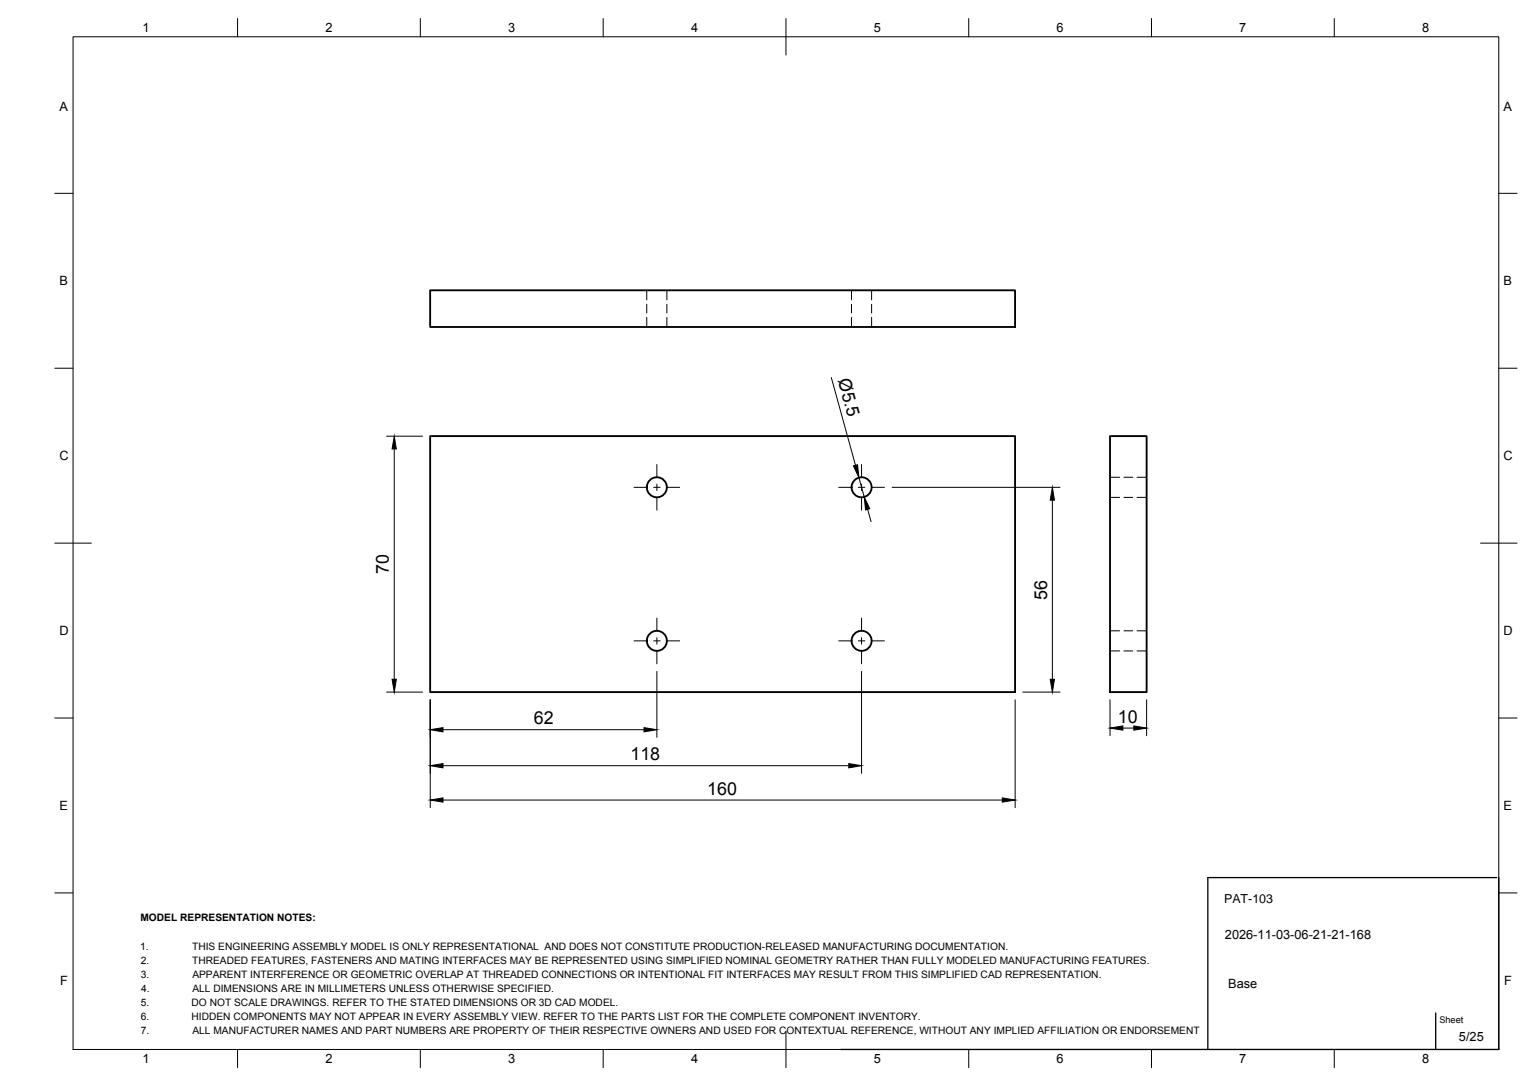
ISO-10303-21;
HEADER;
/* Generated by software containing ST-Developer
 * from STEP Tools, Inc. (www.steptools.com) 
 */

FILE_DESCRIPTION(
/* description */ ('Telescoping shaft support with lock collar'),
/* implementation_level */ '2;1');

FILE_NAME(
/* name */ 'Base.step',
/* time_stamp */ '2026-10-27T10:48:51-07:00',
/* author */ (''),
/* organization */ (''),
/* preprocessor_version */ 'ST-DEVELOPER v20.2',
/* originating_system */ 'Autodesk Translation Framework v15.17.0.0',
/* authorisation */ '');

FILE_SCHEMA (('AUTOMOTIVE_DESIGN { 1 0 10303 214 3 1 1 }'));
ENDSEC;

DATA;
#10=MECHANICAL_DESIGN_GEOMETRIC_PRESENTATION_REPRESENTATION('',(#241),#7349);
#201=SHAPE_REPRESENTATION_RELATIONSHIP('SRR','None',#7443,#221);
#221=ADVANCED_BREP_SHAPE_REPRESENTATION('',(#261),#7327);
#241=STYLED_ITEM('',(#7606),#261);
#261=MANIFOLD_SOLID_BREP('Body1',#3964);
#279=FACE_BOUND('',#730,.T.);
#280=FACE_BOUND('',#731,.T.);
#281=FACE_BOUND('',#732,.T.);
#282=FACE_BOUND('',#733,.T.);
#283=FACE_BOUND('',#735,.T.);
#284=FACE_BOUND('',#736,.T.);
#285=FACE_BOUND('',#737,.T.);
#286=FACE_BOUND('',#738,.T.);
#359=PLANE('',#4222);
#360=PLANE('',#4223);
#361=PLANE('',#4224);
#362=PLANE('',#4225);
#363=PLANE('',#4226);
#364=PLANE('',#4227);
#495=FACE_OUTER_BOUND('',#721,.T.);
#496=FACE_OUTER_BOUND('',#722,.T.);
#497=FACE_OUTER_BOUND('',#723,.T.);
#498=FACE_OUTER_BOUND('',#724,.T.);
#499=FACE_OUTER_BOUND('',#725,.T.);
#500=FACE_OUTER_BOUND('',#726,.T.);
#501=FACE_OUTER_BOUND('',#727,.T.);
#502=FACE_OUTER_BOUND('',#728,.T.);
#503=FACE_OUTER_BOUND('',#729,.T.);
#504=FACE_OUTER_BOUND('',#734,.T.);
#721=EDGE_LOOP('',(#2642,#2643,#2644,#2645));
#722=EDGE_LOOP('',(#2646,#2647,#2648,#2649));
#723=EDGE_LOOP('',(#2650,#2651,#2652,#2653));
#724=EDGE_LOOP('',(#2654,#2655,#2656,#2657));
#725=EDGE_LOOP('',(#2658,#2659,#2660,#2661));
#726=EDGE_LOOP('',(#2662,#2663,#2664,#2665));
#727=EDGE_LOOP('',(#2666,#2667,#2668,#2669));
#728=EDGE_LOOP('',(#2670,#2671,#2672,#2673));
#729=EDGE_LOOP('',(#2674,#2675,#2676,#2677));
#730=EDGE_LOOP('',(#2678));
#731=EDGE_LOOP('',(#2679));
#732=EDGE_LOOP('',(#2680));
#733=EDGE_LOOP('',(#2681));
#734=EDGE_LOOP('',(#2682,#2683,#2684,#2685));
#735=EDGE_LOOP('',(#2686));
#736=EDGE_LOOP('',(#2687));
#737=EDGE_LOOP('',(#2688));
#738=EDGE_LOOP('',(#2689));
#1027=LINE('',#5994,#1307);
#1028=LINE('',#6000,#1308);
#1029=LINE('',#6006,#1309);
#1030=LINE('',#6012,#1310);
#1031=LINE('',#6017,#1311);
#1032=LINE('',#6019,#1312);
#1033=LINE('',#6021,#1313);
#1034=LINE('',#6022,#1314);
#1035=LINE('',#6025,#1315);
#1036=LINE('',#6027,#1316);
#1037=LINE('',#6028,#1317);
#1038=LINE('',#6031,#1318);
#1039=LINE('',#6033,#1319);
#1040=LINE('',#6034,#1320);
#1041=LINE('',#6036,#1321);
#1042=LINE('',#6037,#1322);
#1307=VECTOR('',#4717,0.274999999999999);
#1308=VECTOR('',#4724,0.275);
#1309=VECTOR('',#4731,0.275);
#1310=VECTOR('',#4738,0.274999999999999);
#1311=VECTOR('',#4743,1.);
#1312=VECTOR('',#4744,1.);
#1313=VECTOR('',#4745,1.);
#1314=VECTOR('',#4746,1.);
#1315=VECTOR('',#4749,1.);
#1316=VECTOR('',#4750,1.);
#1317=VECTOR('',#4751,1.);
#1318=VECTOR('',#4754,1.);
#1319=VECTOR('',#4755,1.);
#1320=VECTOR('',#4756,1.);
#1321=VECTOR('',#4759,1.);
#1322=VECTOR('',#4760,1.);
#1587=CIRCLE('',#4211,0.274999999999999);
#1588=CIRCLE('',#4212,0.274999999999999);
#1589=CIRCLE('',#4214,0.275);
#1590=CIRCLE('',#4215,0.275);
#1591=CIRCLE('',#4217,0.275);
#1592=CIRCLE('',#4218,0.275);
#1593=CIRCLE('',#4220,0.274999999999999);
#1594=CIRCLE('',#4221,0.274999999999999);
#1798=VERTEX_POINT('',#5991);
#1799=VERTEX_POINT('',#5993);
#1800=VERTEX_POINT('',#5997);
#1801=VERTEX_POINT('',#5999);
#1802=VERTEX_POINT('',#6003);
#1803=VERTEX_POINT('',#6005);
#1804=VERTEX_POINT('',#6009);
#1805=VERTEX_POINT('',#6011);
#1806=VERTEX_POINT('',#6015);
#1807=VERTEX_POINT('',#6016);
#1808=VERTEX_POINT('',#6018);
#1809=VERTEX_POINT('',#6020);
#1810=VERTEX_POINT('',#6024);
#1811=VERTEX_POINT('',#6026);
#1812=VERTEX_POINT('',#6030);
#1813=VERTEX_POINT('',#6032);
#2133=EDGE_CURVE('',#1798,#1798,#1587,.T.);
#2134=EDGE_CURVE('',#1798,#1799,#1027,.T.);
#2135=EDGE_CURVE('',#1799,#1799,#1588,.T.);
#2136=EDGE_CURVE('',#1800,#1800,#1589,.T.);
#2137=EDGE_CURVE('',#1800,#1801,#1028,.T.);
#2138=EDGE_CURVE('',#1801,#1801,#1590,.T.);
#2139=EDGE_CURVE('',#1802,#1802,#1591,.T.);
#2140=EDGE_CURVE('',#1802,#1803,#1029,.T.);
#2141=EDGE_CURVE('',#1803,#1803,#1592,.T.);
#2142=EDGE_CURVE('',#1804,#1804,#1593,.T.);
#2143=EDGE_CURVE('',#1804,#1805,#1030,.T.);
#2144=EDGE_CURVE('',#1805,#1805,#1594,.T.);
#2145=EDGE_CURVE('',#1806,#1807,#1031,.T.);
#2146=EDGE_CURVE('',#1807,#1808,#1032,.T.);
#2147=EDGE_CURVE('',#1809,#1808,#1033,.T.);
#2148=EDGE_CURVE('',#1806,#1809,#1034,.T.);
#2149=EDGE_CURVE('',#1810,#1806,#1035,.T.);
#2150=EDGE_CURVE('',#1811,#1809,#1036,.T.);
#2151=EDGE_CURVE('',#1810,#1811,#1037,.T.);
#2152=EDGE_CURVE('',#1812,#1810,#1038,.T.);
#2153=EDGE_CURVE('',#1813,#1811,#1039,.T.);
#2154=EDGE_CURVE('',#1812,#1813,#1040,.T.);
#2155=EDGE_CURVE('',#1807,#1812,#1041,.T.);
#2156=EDGE_CURVE('',#1808,#1813,#1042,.T.);
#2642=ORIENTED_EDGE('',*,*,#2133,.F.);
#2643=ORIENTED_EDGE('',*,*,#2134,.T.);
#2644=ORIENTED_EDGE('',*,*,#2135,.F.);
#2645=ORIENTED_EDGE('',*,*,#2134,.F.);
#2646=ORIENTED_EDGE('',*,*,#2136,.F.);
#2647=ORIENTED_EDGE('',*,*,#2137,.T.);
#2648=ORIENTED_EDGE('',*,*,#2138,.F.);
#2649=ORIENTED_EDGE('',*,*,#2137,.F.);
#2650=ORIENTED_EDGE('',*,*,#2139,.F.);
#2651=ORIENTED_EDGE('',*,*,#2140,.T.);
#2652=ORIENTED_EDGE('',*,*,#2141,.F.);
#2653=ORIENTED_EDGE('',*,*,#2140,.F.);
#2654=ORIENTED_EDGE('',*,*,#2142,.F.);
#2655=ORIENTED_EDGE('',*,*,#2143,.T.);
#2656=ORIENTED_EDGE('',*,*,#2144,.F.);
#2657=ORIENTED_EDGE('',*,*,#2143,.F.);
#2658=ORIENTED_EDGE('',*,*,#2145,.T.);
#2659=ORIENTED_EDGE('',*,*,#2146,.T.);
#2660=ORIENTED_EDGE('',*,*,#2147,.F.);
#2661=ORIENTED_EDGE('',*,*,#2148,.F.);
#2662=ORIENTED_EDGE('',*,*,#2149,.T.);
#2663=ORIENTED_EDGE('',*,*,#2148,.T.);
#2664=ORIENTED_EDGE('',*,*,#2150,.F.);
#2665=ORIENTED_EDGE('',*,*,#2151,.F.);
#2666=ORIENTED_EDGE('',*,*,#2152,.T.);
#2667=ORIENTED_EDGE('',*,*,#2151,.T.);
#2668=ORIENTED_EDGE('',*,*,#2153,.F.);
#2669=ORIENTED_EDGE('',*,*,#2154,.F.);
#2670=ORIENTED_EDGE('',*,*,#2155,.T.);
#2671=ORIENTED_EDGE('',*,*,#2154,.T.);
#2672=ORIENTED_EDGE('',*,*,#2156,.F.);
#2673=ORIENTED_EDGE('',*,*,#2146,.F.);
#2674=ORIENTED_EDGE('',*,*,#2156,.T.);
#2675=ORIENTED_EDGE('',*,*,#2153,.T.);
#2676=ORIENTED_EDGE('',*,*,#2150,.T.);
#2677=ORIENTED_EDGE('',*,*,#2147,.T.);
#2678=ORIENTED_EDGE('',*,*,#2135,.T.);
#2679=ORIENTED_EDGE('',*,*,#2138,.T.);
#2680=ORIENTED_EDGE('',*,*,#2141,.T.);
#2681=ORIENTED_EDGE('',*,*,#2144,.T.);
#2682=ORIENTED_EDGE('',*,*,#2155,.F.);
#2683=ORIENTED_EDGE('',*,*,#2145,.F.);
#2684=ORIENTED_EDGE('',*,*,#2149,.F.);
#2685=ORIENTED_EDGE('',*,*,#2152,.F.);
#2686=ORIENTED_EDGE('',*,*,#2133,.T.);
#2687=ORIENTED_EDGE('',*,*,#2136,.T.);
#2688=ORIENTED_EDGE('',*,*,#2139,.T.);
#2689=ORIENTED_EDGE('',*,*,#2142,.T.);
#3660=CYLINDRICAL_SURFACE('',#4210,0.274999999999999);
#3661=CYLINDRICAL_SURFACE('',#4213,0.275);
#3662=CYLINDRICAL_SURFACE('',#4216,0.275);
#3663=CYLINDRICAL_SURFACE('',#4219,0.274999999999999);
#3738=ADVANCED_FACE('',(#495),#3660,.F.);
#3739=ADVANCED_FACE('',(#496),#3661,.F.);
#3740=ADVANCED_FACE('',(#497),#3662,.F.);
#3741=ADVANCED_FACE('',(#498),#3663,.F.);
#3742=ADVANCED_FACE('',(#499),#359,.T.);
#3743=ADVANCED_FACE('',(#500),#360,.T.);
#3744=ADVANCED_FACE('',(#501),#361,.T.);
#3745=ADVANCED_FACE('',(#502),#362,.T.);
#3746=ADVANCED_FACE('',(#503,#279,#280,#281,#282),#363,.T.);
#3747=ADVANCED_FACE('',(#504,#283,#284,#285,#286),#364,.F.);
#3964=CLOSED_SHELL('',(#3738,#3739,#3740,#3741,#3742,#3743,#3744,#3745,
#3746,#3747));
#4209=AXIS2_PLACEMENT_3D('',#5989,#4711,#4712);
#4210=AXIS2_PLACEMENT_3D('',#5990,#4713,#4714);
#4211=AXIS2_PLACEMENT_3D('',#5992,#4715,#4716);
#4212=AXIS2_PLACEMENT_3D('',#5995,#4718,#4719);
#4213=AXIS2_PLACEMENT_3D('',#5996,#4720,#4721);
#4214=AXIS2_PLACEMENT_3D('',#5998,#4722,#4723);
#4215=AXIS2_PLACEMENT_3D('',#6001,#4725,#4726);
#4216=AXIS2_PLACEMENT_3D('',#6002,#4727,#4728);
#4217=AXIS2_PLACEMENT_3D('',#6004,#4729,#4730);
#4218=AXIS2_PLACEMENT_3D('',#6007,#4732,#4733);
#4219=AXIS2_PLACEMENT_3D('',#6008,#4734,#4735);
#4220=AXIS2_PLACEMENT_3D('',#6010,#4736,#4737);
#4221=AXIS2_PLACEMENT_3D('',#6013,#4739,#4740);
#4222=AXIS2_PLACEMENT_3D('',#6014,#4741,#4742);
#4223=AXIS2_PLACEMENT_3D('',#6023,#4747,#4748);
#4224=AXIS2_PLACEMENT_3D('',#6029,#4752,#4753);
#4225=AXIS2_PLACEMENT_3D('',#6035,#4757,#4758);
#4226=AXIS2_PLACEMENT_3D('',#6038,#4761,#4762);
#4227=AXIS2_PLACEMENT_3D('',#6039,#4763,#4764);
#4711=DIRECTION('axis',(0.,0.,1.));
#4712=DIRECTION('refdir',(1.,0.,0.));
#4713=DIRECTION('center_axis',(0.,0.,1.));
#4714=DIRECTION('ref_axis',(1.,0.,0.));
#4715=DIRECTION('center_axis',(0.,0.,1.));
#4716=DIRECTION('ref_axis',(1.,0.,0.));
#4717=DIRECTION('',(0.,0.,1.));
#4718=DIRECTION('center_axis',(0.,0.,-1.));
#4719=DIRECTION('ref_axis',(1.,0.,0.));
#4720=DIRECTION('center_axis',(0.,0.,1.));
#4721=DIRECTION('ref_axis',(1.,0.,0.));
#4722=DIRECTION('center_axis',(0.,0.,1.));
#4723=DIRECTION('ref_axis',(1.,0.,0.));
#4724=DIRECTION('',(0.,0.,1.));
#4725=DIRECTION('center_axis',(0.,0.,-1.));
#4726=DIRECTION('ref_axis',(1.,0.,0.));
#4727=DIRECTION('center_axis',(0.,0.,1.));
#4728=DIRECTION('ref_axis',(1.,0.,0.));
#4729=DIRECTION('center_axis',(0.,0.,1.));
#4730=DIRECTION('ref_axis',(1.,0.,0.));
#4731=DIRECTION('',(0.,0.,1.));
#4732=DIRECTION('center_axis',(0.,0.,-1.));
#4733=DIRECTION('ref_axis',(1.,0.,0.));
#4734=DIRECTION('center_axis',(0.,0.,1.));
#4735=DIRECTION('ref_axis',(1.,0.,0.));
#4736=DIRECTION('center_axis',(0.,0.,1.));
#4737=DIRECTION('ref_axis',(1.,0.,0.));
#4738=DIRECTION('',(0.,0.,1.));
#4739=DIRECTION('center_axis',(0.,0.,-1.));
#4740=DIRECTION('ref_axis',(1.,0.,0.));
#4741=DIRECTION('center_axis',(0.,1.,0.));
#4742=DIRECTION('ref_axis',(-1.,0.,0.));
#4743=DIRECTION('',(-1.,0.,0.));
#4744=DIRECTION('',(0.,0.,1.));
#4745=DIRECTION('',(-1.,0.,0.));
#4746=DIRECTION('',(0.,0.,1.));
#4747=DIRECTION('center_axis',(1.,0.,0.));
#4748=DIRECTION('ref_axis',(0.,1.,0.));
#4749=DIRECTION('',(0.,1.,0.));
#4750=DIRECTION('',(0.,1.,0.));
#4751=DIRECTION('',(0.,0.,1.));
#4752=DIRECTION('center_axis',(0.,-1.,0.));
#4753=DIRECTION('ref_axis',(1.,0.,0.));
#4754=DIRECTION('',(1.,0.,0.));
#4755=DIRECTION('',(1.,0.,0.));
#4756=DIRECTION('',(0.,0.,1.));
#4757=DIRECTION('center_axis',(-1.,0.,0.));
#4758=DIRECTION('ref_axis',(0.,-1.,0.));
#4759=DIRECTION('',(0.,-1.,0.));
#4760=DIRECTION('',(0.,-1.,0.));
#4761=DIRECTION('center_axis',(0.,0.,1.));
#4762=DIRECTION('ref_axis',(1.,0.,0.));
#4763=DIRECTION('center_axis',(0.,0.,1.));
#4764=DIRECTION('ref_axis',(1.,0.,0.));
#5989=CARTESIAN_POINT('',(0.,0.,0.));
#5990=CARTESIAN_POINT('Origin',(7.8,-2.1,-0.1));
#5991=CARTESIAN_POINT('',(7.525,-2.1,0.));
#5992=CARTESIAN_POINT('Origin',(7.8,-2.1,0.));
#5993=CARTESIAN_POINT('',(7.525,-2.1,1.));
#5994=CARTESIAN_POINT('',(7.525,-2.1,-0.1));
#5995=CARTESIAN_POINT('Origin',(7.8,-2.1,1.));
#5996=CARTESIAN_POINT('Origin',(2.2,2.1,-0.1));
#5997=CARTESIAN_POINT('',(1.925,2.1,0.));
#5998=CARTESIAN_POINT('Origin',(2.2,2.1,0.));
#5999=CARTESIAN_POINT('',(1.925,2.1,1.));
#6000=CARTESIAN_POINT('',(1.925,2.1,-0.1));
#6001=CARTESIAN_POINT('Origin',(2.2,2.1,1.));
#6002=CARTESIAN_POINT('Origin',(2.2,-2.1,-0.1));
#6003=CARTESIAN_POINT('',(1.925,-2.1,0.));
#6004=CARTESIAN_POINT('Origin',(2.2,-2.1,0.));
#6005=CARTESIAN_POINT('',(1.925,-2.1,1.));
#6006=CARTESIAN_POINT('',(1.925,-2.1,-0.1));
#6007=CARTESIAN_POINT('Origin',(2.2,-2.1,1.));
#6008=CARTESIAN_POINT('Origin',(7.8,2.1,-0.1));
#6009=CARTESIAN_POINT('',(7.525,2.1,0.));
#6010=CARTESIAN_POINT('Origin',(7.8,2.1,0.));
#6011=CARTESIAN_POINT('',(7.525,2.1,1.));
#6012=CARTESIAN_POINT('',(7.525,2.1,-0.1));
#6013=CARTESIAN_POINT('Origin',(7.8,2.1,1.));
#6014=CARTESIAN_POINT('Origin',(14.,3.5,0.));
#6015=CARTESIAN_POINT('',(14.,3.5,0.));
#6016=CARTESIAN_POINT('',(-2.,3.5,0.));
#6017=CARTESIAN_POINT('',(14.,3.5,0.));
#6018=CARTESIAN_POINT('',(-2.,3.5,1.));
#6019=CARTESIAN_POINT('',(-2.,3.5,0.));
#6020=CARTESIAN_POINT('',(14.,3.5,1.));
#6021=CARTESIAN_POINT('',(14.,3.5,1.));
#6022=CARTESIAN_POINT('',(14.,3.5,0.));
#6023=CARTESIAN_POINT('Origin',(14.,-3.5,0.));
#6024=CARTESIAN_POINT('',(14.,-3.5,0.));
#6025=CARTESIAN_POINT('',(14.,-3.5,0.));
#6026=CARTESIAN_POINT('',(14.,-3.5,1.));
#6027=CARTESIAN_POINT('',(14.,-3.5,1.));
#6028=CARTESIAN_POINT('',(14.,-3.5,0.));
#6029=CARTESIAN_POINT('Origin',(-2.,-3.5,0.));
#6030=CARTESIAN_POINT('',(-2.,-3.5,0.));
#6031=CARTESIAN_POINT('',(-2.,-3.5,0.));
#6032=CARTESIAN_POINT('',(-2.,-3.5,1.));
#6033=CARTESIAN_POINT('',(-2.,-3.5,1.));
#6034=CARTESIAN_POINT('',(-2.,-3.5,0.));
#6035=CARTESIAN_POINT('Origin',(-2.,3.5,0.));
#6036=CARTESIAN_POINT('',(-2.,3.5,0.));
#6037=CARTESIAN_POINT('',(-2.,3.5,1.));
#6038=CARTESIAN_POINT('Origin',(6.,0.,1.));
#6039=CARTESIAN_POINT('Origin',(6.,0.,0.));
#7302=UNCERTAINTY_MEASURE_WITH_UNIT(LENGTH_MEASURE(0.001),#7350,
'DISTANCE_ACCURACY_VALUE',
'Maximum model space distance between geometric entities at asserted c
onnectivities');
#7324=UNCERTAINTY_MEASURE_WITH_UNIT(LENGTH_MEASURE(0.001),#7350,
'DISTANCE_ACCURACY_VALUE',
'Maximum model space distance between geometric entities at asserted c
onnectivities');
#7327=(
GEOMETRIC_REPRESENTATION_CONTEXT(3)
GLOBAL_UNCERTAINTY_ASSIGNED_CONTEXT((#7302))
GLOBAL_UNIT_ASSIGNED_CONTEXT((#7350,#7352,#7353))
REPRESENTATION_CONTEXT('','3D')
);
#7349=(
GEOMETRIC_REPRESENTATION_CONTEXT(3)
GLOBAL_UNCERTAINTY_ASSIGNED_CONTEXT((#7324))
GLOBAL_UNIT_ASSIGNED_CONTEXT((#7350,#7352,#7353))
REPRESENTATION_CONTEXT('','3D')
);
#7350=(
LENGTH_UNIT()
NAMED_UNIT(*)
SI_UNIT(.CENTI.,.METRE.)
);
#7352=(
NAMED_UNIT(*)
PLANE_ANGLE_UNIT()
SI_UNIT($,.RADIAN.)
);
#7353=(
NAMED_UNIT(*)
SI_UNIT($,.STERADIAN.)
SOLID_ANGLE_UNIT()
);
#7356=SHAPE_DEFINITION_REPRESENTATION(#7380,#7443);
#7380=PRODUCT_DEFINITION_SHAPE('',$,#7468);
#7443=SHAPE_REPRESENTATION('',(#4209),#7327);
#7465=PRODUCT_DEFINITION_CONTEXT('part definition',#7539,'design');
#7468=PRODUCT_DEFINITION('Base','Base',#7492,#7465);
#7492=PRODUCT_DEFINITION_FORMATION('',$,#7543);
#7539=APPLICATION_CONTEXT(
'Core Data for Automotive Mechanical Design Process');
#7540=PRODUCT_CONTEXT('part definition',#7539,'mechanical');
#7543=PRODUCT('Base','Base','Base',(#7540));
#7600=COLOUR_RGB('Dark Blue',0.08,0.2,0.34);
#7601=FILL_AREA_STYLE_COLOUR('',#7600);
#7602=FILL_AREA_STYLE('',(#7601));
#7603=SURFACE_STYLE_FILL_AREA(#7602);
#7604=SURFACE_SIDE_STYLE('',(#7603));
#7605=SURFACE_STYLE_USAGE(.BOTH.,#7604);
#7606=PRESENTATION_STYLE_ASSIGNMENT((#7605));
ENDSEC;
END-ISO-10303-21;
